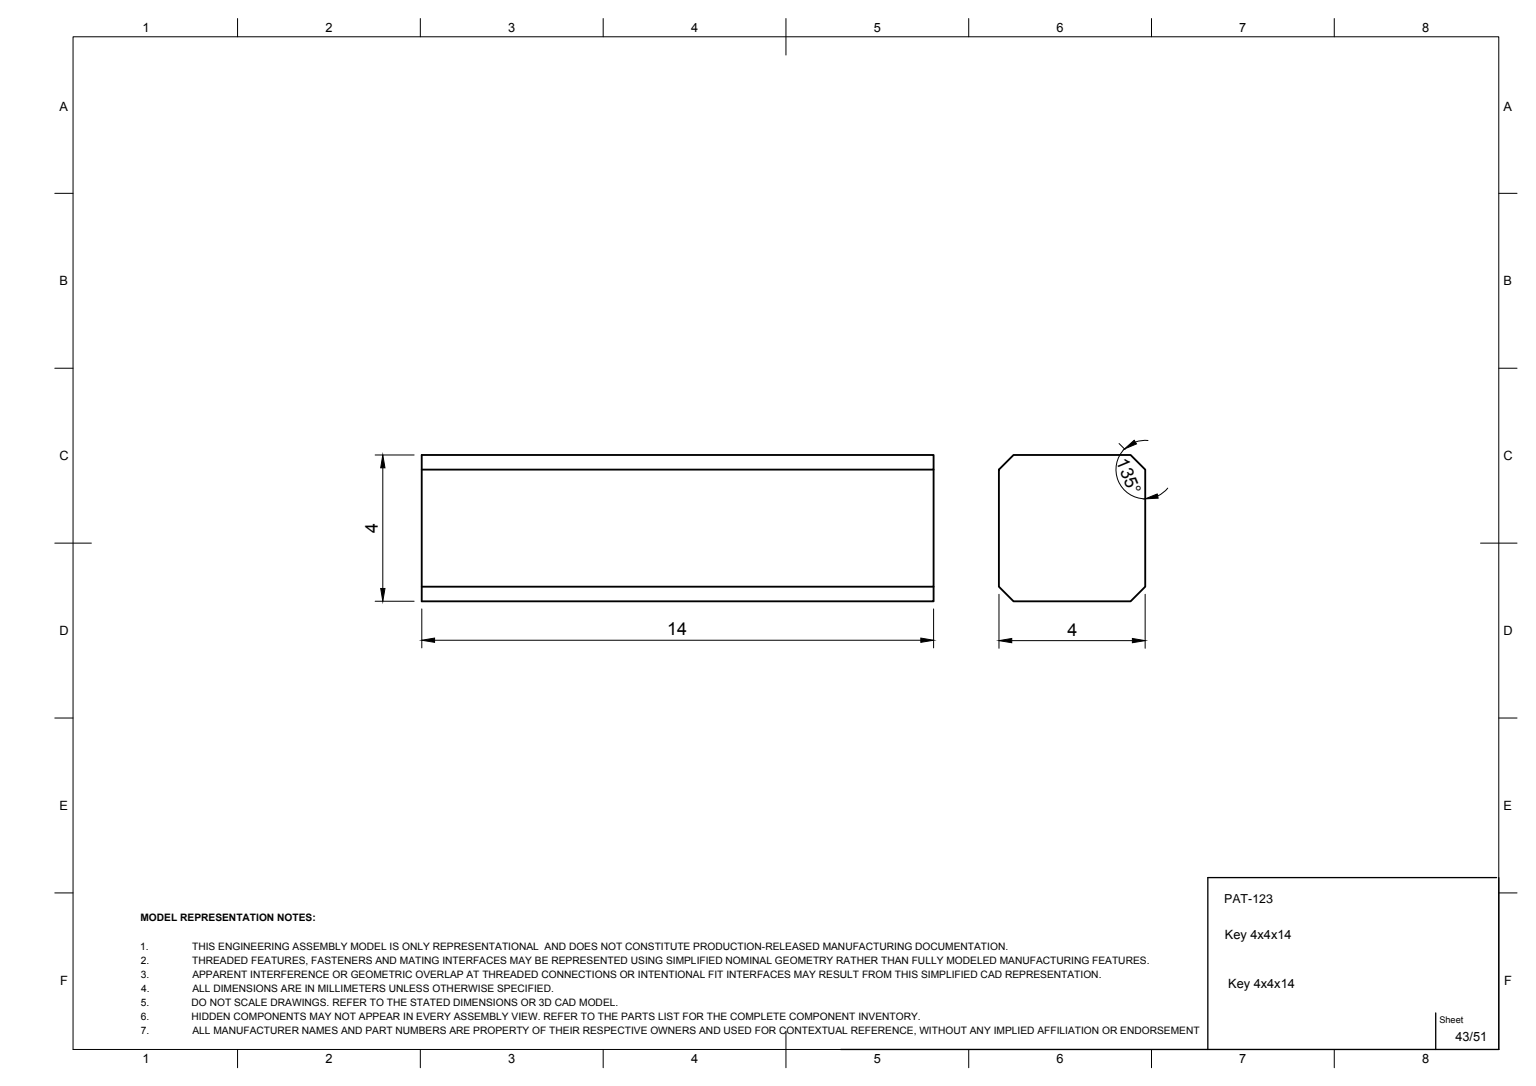
ISO-10303-21;
HEADER;
/* Generated by software containing ST-Developer
 * from STEP Tools, Inc. (www.steptools.com) 
 */

FILE_DESCRIPTION(
/* description */ ('Worm-less right-angle friction wheel drive'),
/* implementation_level */ '2;1');

FILE_NAME(
/* name */ 'Key 4x4x14.step',
/* time_stamp */ '2026-10-28T03:22:36-07:00',
/* author */ (''),
/* organization */ (''),
/* preprocessor_version */ 'ST-DEVELOPER v20.2',
/* originating_system */ 'Autodesk Translation Framework v15.17.0.0',
/* authorisation */ '');

FILE_SCHEMA (('AUTOMOTIVE_DESIGN { 1 0 10303 214 3 1 1 }'));
ENDSEC;

DATA;
#10=MECHANICAL_DESIGN_GEOMETRIC_PRESENTATION_REPRESENTATION('',(#663),#17046);
#562=SHAPE_REPRESENTATION_RELATIONSHIP('SRR','None',#17308,#609);
#609=ADVANCED_BREP_SHAPE_REPRESENTATION('',(#713),#17044);
#663=STYLED_ITEM('',(#17591),#713);
#713=MANIFOLD_SOLID_BREP('Body1',#8222);
#1189=PLANE('',#9727);
#1190=PLANE('',#9728);
#1191=PLANE('',#9729);
#1192=PLANE('',#9730);
#1193=PLANE('',#9731);
#1194=PLANE('',#9732);
#1195=PLANE('',#9733);
#1196=PLANE('',#9734);
#1197=PLANE('',#9735);
#1198=PLANE('',#9736);
#1653=FACE_OUTER_BOUND('',#2355,.T.);
#1654=FACE_OUTER_BOUND('',#2356,.T.);
#1655=FACE_OUTER_BOUND('',#2357,.T.);
#1656=FACE_OUTER_BOUND('',#2358,.T.);
#1657=FACE_OUTER_BOUND('',#2359,.T.);
#1658=FACE_OUTER_BOUND('',#2360,.T.);
#1659=FACE_OUTER_BOUND('',#2361,.T.);
#1660=FACE_OUTER_BOUND('',#2362,.T.);
#1661=FACE_OUTER_BOUND('',#2363,.T.);
#1662=FACE_OUTER_BOUND('',#2364,.T.);
#2355=EDGE_LOOP('',(#7436,#7437,#7438,#7439,#7440,#7441,#7442,#7443));
#2356=EDGE_LOOP('',(#7444,#7445,#7446,#7447));
#2357=EDGE_LOOP('',(#7448,#7449,#7450,#7451));
#2358=EDGE_LOOP('',(#7452,#7453,#7454,#7455));
#2359=EDGE_LOOP('',(#7456,#7457,#7458,#7459));
#2360=EDGE_LOOP('',(#7460,#7461,#7462,#7463,#7464,#7465,#7466,#7467));
#2361=EDGE_LOOP('',(#7468,#7469,#7470,#7471));
#2362=EDGE_LOOP('',(#7472,#7473,#7474,#7475));
#2363=EDGE_LOOP('',(#7476,#7477,#7478,#7479));
#2364=EDGE_LOOP('',(#7480,#7481,#7482,#7483));
#2873=LINE('',#16823,#3413);
#2874=LINE('',#16825,#3414);
#2875=LINE('',#16827,#3415);
#2876=LINE('',#16829,#3416);
#2877=LINE('',#16831,#3417);
#2878=LINE('',#16833,#3418);
#2879=LINE('',#16835,#3419);
#2880=LINE('',#16836,#3420);
#2881=LINE('',#16839,#3421);
#2882=LINE('',#16841,#3422);
#2883=LINE('',#16842,#3423);
#2884=LINE('',#16845,#3424);
#2885=LINE('',#16846,#3425);
#2886=LINE('',#16849,#3426);
#2887=LINE('',#16850,#3427);
#2888=LINE('',#16853,#3428);
#2889=LINE('',#16854,#3429);
#2890=LINE('',#16857,#3430);
#2891=LINE('',#16859,#3431);
#2892=LINE('',#16861,#3432);
#2893=LINE('',#16862,#3433);
#2894=LINE('',#16864,#3434);
#2895=LINE('',#16866,#3435);
#2896=LINE('',#16868,#3436);
#3413=VECTOR('',#12241,1.);
#3414=VECTOR('',#12242,1.);
#3415=VECTOR('',#12243,1.);
#3416=VECTOR('',#12244,1.);
#3417=VECTOR('',#12245,1.);
#3418=VECTOR('',#12246,1.);
#3419=VECTOR('',#12247,1.);
#3420=VECTOR('',#12248,1.);
#3421=VECTOR('',#12251,1.);
#3422=VECTOR('',#12252,1.);
#3423=VECTOR('',#12253,1.);
#3424=VECTOR('',#12256,1.);
#3425=VECTOR('',#12257,1.);
#3426=VECTOR('',#12260,1.);
#3427=VECTOR('',#12261,1.);
#3428=VECTOR('',#12264,1.);
#3429=VECTOR('',#12265,1.);
#3430=VECTOR('',#12268,1.);
#3431=VECTOR('',#12269,1.);
#3432=VECTOR('',#12270,1.);
#3433=VECTOR('',#12271,1.);
#3434=VECTOR('',#12274,1.);
#3435=VECTOR('',#12277,1.);
#3436=VECTOR('',#12280,1.);
#4505=VERTEX_POINT('',#16821);
#4506=VERTEX_POINT('',#16822);
#4507=VERTEX_POINT('',#16824);
#4508=VERTEX_POINT('',#16826);
#4509=VERTEX_POINT('',#16828);
#4510=VERTEX_POINT('',#16830);
#4511=VERTEX_POINT('',#16832);
#4512=VERTEX_POINT('',#16834);
#4513=VERTEX_POINT('',#16838);
#4514=VERTEX_POINT('',#16840);
#4515=VERTEX_POINT('',#16844);
#4516=VERTEX_POINT('',#16848);
#4517=VERTEX_POINT('',#16852);
#4518=VERTEX_POINT('',#16856);
#4519=VERTEX_POINT('',#16858);
#4520=VERTEX_POINT('',#16860);
#5487=EDGE_CURVE('',#4505,#4506,#2873,.T.);
#5488=EDGE_CURVE('',#4507,#4505,#2874,.T.);
#5489=EDGE_CURVE('',#4508,#4507,#2875,.T.);
#5490=EDGE_CURVE('',#4509,#4508,#2876,.T.);
#5491=EDGE_CURVE('',#4510,#4509,#2877,.T.);
#5492=EDGE_CURVE('',#4511,#4510,#2878,.T.);
#5493=EDGE_CURVE('',#4512,#4511,#2879,.T.);
#5494=EDGE_CURVE('',#4506,#4512,#2880,.T.);
#5495=EDGE_CURVE('',#4509,#4513,#2881,.T.);
#5496=EDGE_CURVE('',#4513,#4514,#2882,.T.);
#5497=EDGE_CURVE('',#4514,#4510,#2883,.T.);
#5498=EDGE_CURVE('',#4515,#4508,#2884,.T.);
#5499=EDGE_CURVE('',#4515,#4513,#2885,.T.);
#5500=EDGE_CURVE('',#4507,#4516,#2886,.T.);
#5501=EDGE_CURVE('',#4516,#4515,#2887,.T.);
#5502=EDGE_CURVE('',#4517,#4505,#2888,.T.);
#5503=EDGE_CURVE('',#4517,#4516,#2889,.T.);
#5504=EDGE_CURVE('',#4518,#4517,#2890,.T.);
#5505=EDGE_CURVE('',#4519,#4518,#2891,.T.);
#5506=EDGE_CURVE('',#4520,#4519,#2892,.T.);
#5507=EDGE_CURVE('',#4514,#4520,#2893,.T.);
#5508=EDGE_CURVE('',#4506,#4518,#2894,.T.);
#5509=EDGE_CURVE('',#4519,#4512,#2895,.T.);
#5510=EDGE_CURVE('',#4511,#4520,#2896,.T.);
#7436=ORIENTED_EDGE('',*,*,#5487,.F.);
#7437=ORIENTED_EDGE('',*,*,#5488,.F.);
#7438=ORIENTED_EDGE('',*,*,#5489,.F.);
#7439=ORIENTED_EDGE('',*,*,#5490,.F.);
#7440=ORIENTED_EDGE('',*,*,#5491,.F.);
#7441=ORIENTED_EDGE('',*,*,#5492,.F.);
#7442=ORIENTED_EDGE('',*,*,#5493,.F.);
#7443=ORIENTED_EDGE('',*,*,#5494,.F.);
#7444=ORIENTED_EDGE('',*,*,#5491,.T.);
#7445=ORIENTED_EDGE('',*,*,#5495,.T.);
#7446=ORIENTED_EDGE('',*,*,#5496,.T.);
#7447=ORIENTED_EDGE('',*,*,#5497,.T.);
#7448=ORIENTED_EDGE('',*,*,#5490,.T.);
#7449=ORIENTED_EDGE('',*,*,#5498,.F.);
#7450=ORIENTED_EDGE('',*,*,#5499,.T.);
#7451=ORIENTED_EDGE('',*,*,#5495,.F.);
#7452=ORIENTED_EDGE('',*,*,#5489,.T.);
#7453=ORIENTED_EDGE('',*,*,#5500,.T.);
#7454=ORIENTED_EDGE('',*,*,#5501,.T.);
#7455=ORIENTED_EDGE('',*,*,#5498,.T.);
#7456=ORIENTED_EDGE('',*,*,#5488,.T.);
#7457=ORIENTED_EDGE('',*,*,#5502,.F.);
#7458=ORIENTED_EDGE('',*,*,#5503,.T.);
#7459=ORIENTED_EDGE('',*,*,#5500,.F.);
#7460=ORIENTED_EDGE('',*,*,#5496,.F.);
#7461=ORIENTED_EDGE('',*,*,#5499,.F.);
#7462=ORIENTED_EDGE('',*,*,#5501,.F.);
#7463=ORIENTED_EDGE('',*,*,#5503,.F.);
#7464=ORIENTED_EDGE('',*,*,#5504,.F.);
#7465=ORIENTED_EDGE('',*,*,#5505,.F.);
#7466=ORIENTED_EDGE('',*,*,#5506,.F.);
#7467=ORIENTED_EDGE('',*,*,#5507,.F.);
#7468=ORIENTED_EDGE('',*,*,#5487,.T.);
#7469=ORIENTED_EDGE('',*,*,#5508,.T.);
#7470=ORIENTED_EDGE('',*,*,#5504,.T.);
#7471=ORIENTED_EDGE('',*,*,#5502,.T.);
#7472=ORIENTED_EDGE('',*,*,#5494,.T.);
#7473=ORIENTED_EDGE('',*,*,#5509,.F.);
#7474=ORIENTED_EDGE('',*,*,#5505,.T.);
#7475=ORIENTED_EDGE('',*,*,#5508,.F.);
#7476=ORIENTED_EDGE('',*,*,#5493,.T.);
#7477=ORIENTED_EDGE('',*,*,#5510,.T.);
#7478=ORIENTED_EDGE('',*,*,#5506,.T.);
#7479=ORIENTED_EDGE('',*,*,#5509,.T.);
#7480=ORIENTED_EDGE('',*,*,#5492,.T.);
#7481=ORIENTED_EDGE('',*,*,#5497,.F.);
#7482=ORIENTED_EDGE('',*,*,#5507,.T.);
#7483=ORIENTED_EDGE('',*,*,#5510,.F.);
#8145=ADVANCED_FACE('',(#1653),#1189,.T.);
#8146=ADVANCED_FACE('',(#1654),#1190,.T.);
#8147=ADVANCED_FACE('',(#1655),#1191,.T.);
#8148=ADVANCED_FACE('',(#1656),#1192,.T.);
#8149=ADVANCED_FACE('',(#1657),#1193,.T.);
#8150=ADVANCED_FACE('',(#1658),#1194,.F.);
#8151=ADVANCED_FACE('',(#1659),#1195,.T.);
#8152=ADVANCED_FACE('',(#1660),#1196,.T.);
#8153=ADVANCED_FACE('',(#1661),#1197,.T.);
#8154=ADVANCED_FACE('',(#1662),#1198,.F.);
#8222=CLOSED_SHELL('',(#8145,#8146,#8147,#8148,#8149,#8150,#8151,#8152,
#8153,#8154));
#9726=AXIS2_PLACEMENT_3D('',#16819,#12237,#12238);
#9727=AXIS2_PLACEMENT_3D('',#16820,#12239,#12240);
#9728=AXIS2_PLACEMENT_3D('',#16837,#12249,#12250);
#9729=AXIS2_PLACEMENT_3D('',#16843,#12254,#12255);
#9730=AXIS2_PLACEMENT_3D('',#16847,#12258,#12259);
#9731=AXIS2_PLACEMENT_3D('',#16851,#12262,#12263);
#9732=AXIS2_PLACEMENT_3D('',#16855,#12266,#12267);
#9733=AXIS2_PLACEMENT_3D('',#16863,#12272,#12273);
#9734=AXIS2_PLACEMENT_3D('',#16865,#12275,#12276);
#9735=AXIS2_PLACEMENT_3D('',#16867,#12278,#12279);
#9736=AXIS2_PLACEMENT_3D('',#16869,#12281,#12282);
#12237=DIRECTION('axis',(0.,0.,1.));
#12238=DIRECTION('refdir',(1.,0.,0.));
#12239=DIRECTION('center_axis',(1.,0.,0.));
#12240=DIRECTION('ref_axis',(0.,0.,-1.));
#12241=DIRECTION('',(0.,0.707106781186547,-0.707106781186548));
#12242=DIRECTION('',(0.,1.,0.));
#12243=DIRECTION('',(0.,0.707106781186547,0.707106781186548));
#12244=DIRECTION('',(0.,0.,1.));
#12245=DIRECTION('',(0.,-0.707106781186548,0.707106781186548));
#12246=DIRECTION('',(0.,-1.,0.));
#12247=DIRECTION('',(0.,-0.707106781186548,-0.707106781186548));
#12248=DIRECTION('',(0.,0.,-1.));
#12249=DIRECTION('center_axis',(0.,-0.707106781186548,-0.707106781186548));
#12250=DIRECTION('ref_axis',(-1.,0.,0.));
#12251=DIRECTION('',(-1.,0.,0.));
#12252=DIRECTION('',(0.,0.707106781186548,-0.707106781186548));
#12253=DIRECTION('',(1.,0.,0.));
#12254=DIRECTION('center_axis',(0.,-1.,0.));
#12255=DIRECTION('ref_axis',(1.,0.,0.));
#12256=DIRECTION('',(1.,0.,0.));
#12257=DIRECTION('',(0.,0.,-1.));
#12258=DIRECTION('center_axis',(0.,-0.707106781186548,0.707106781186547));
#12259=DIRECTION('ref_axis',(1.,0.,0.));
#12260=DIRECTION('',(-1.,0.,0.));
#12261=DIRECTION('',(0.,-0.707106781186547,-0.707106781186548));
#12262=DIRECTION('center_axis',(0.,0.,1.));
#12263=DIRECTION('ref_axis',(1.,0.,0.));
#12264=DIRECTION('',(1.,0.,0.));
#12265=DIRECTION('',(0.,-1.,0.));
#12266=DIRECTION('center_axis',(1.,0.,0.));
#12267=DIRECTION('ref_axis',(0.,0.,-1.));
#12268=DIRECTION('',(0.,-0.707106781186547,0.707106781186548));
#12269=DIRECTION('',(0.,0.,1.));
#12270=DIRECTION('',(0.,0.707106781186548,0.707106781186548));
#12271=DIRECTION('',(0.,1.,0.));
#12272=DIRECTION('center_axis',(0.,0.707106781186548,0.707106781186547));
#12273=DIRECTION('ref_axis',(1.,0.,0.));
#12274=DIRECTION('',(-1.,0.,0.));
#12275=DIRECTION('center_axis',(0.,1.,0.));
#12276=DIRECTION('ref_axis',(-1.,0.,0.));
#12277=DIRECTION('',(1.,0.,0.));
#12278=DIRECTION('center_axis',(0.,0.707106781186548,-0.707106781186548));
#12279=DIRECTION('ref_axis',(-1.,0.,0.));
#12280=DIRECTION('',(-1.,0.,0.));
#12281=DIRECTION('center_axis',(0.,0.,1.));
#12282=DIRECTION('ref_axis',(1.,0.,0.));
#16819=CARTESIAN_POINT('',(0.,0.,0.));
#16820=CARTESIAN_POINT('Origin',(0.7,0.,0.25));
#16821=CARTESIAN_POINT('',(0.7,0.16,0.4));
#16822=CARTESIAN_POINT('',(0.7,0.2,0.36));
#16823=CARTESIAN_POINT('',(0.7,0.1675,0.3925));
#16824=CARTESIAN_POINT('',(0.7,-0.16,0.4));
#16825=CARTESIAN_POINT('',(0.7,0.,0.4));
#16826=CARTESIAN_POINT('',(0.7,-0.2,0.36));
#16827=CARTESIAN_POINT('',(0.7,-0.1675,0.3925));
#16828=CARTESIAN_POINT('',(0.7,-0.2,0.04));
#16829=CARTESIAN_POINT('',(0.7,-0.2,0.125));
#16830=CARTESIAN_POINT('',(0.7,-0.16,0.));
#16831=CARTESIAN_POINT('',(0.7,-0.1925,0.0325));
#16832=CARTESIAN_POINT('',(0.7,0.16,0.));
#16833=CARTESIAN_POINT('',(0.7,0.,0.));
#16834=CARTESIAN_POINT('',(0.7,0.2,0.04));
#16835=CARTESIAN_POINT('',(0.7,0.1925,0.0325));
#16836=CARTESIAN_POINT('',(0.7,0.2,0.125));
#16837=CARTESIAN_POINT('Origin',(-0.4,-0.18,0.02));
#16838=CARTESIAN_POINT('',(-0.7,-0.2,0.04));
#16839=CARTESIAN_POINT('',(-0.4,-0.2,0.04));
#16840=CARTESIAN_POINT('',(-0.7,-0.16,0.));
#16841=CARTESIAN_POINT('',(-0.7,-0.1925,0.0325));
#16842=CARTESIAN_POINT('',(-0.4,-0.16,0.));
#16843=CARTESIAN_POINT('Origin',(-0.8,-0.2,0.));
#16844=CARTESIAN_POINT('',(-0.7,-0.2,0.36));
#16845=CARTESIAN_POINT('',(-0.4,-0.2,0.36));
#16846=CARTESIAN_POINT('',(-0.7,-0.2,0.125));
#16847=CARTESIAN_POINT('Origin',(-0.4,-0.18,0.38));
#16848=CARTESIAN_POINT('',(-0.7,-0.16,0.4));
#16849=CARTESIAN_POINT('',(-0.4,-0.16,0.4));
#16850=CARTESIAN_POINT('',(-0.7,-0.1675,0.3925));
#16851=CARTESIAN_POINT('Origin',(0.,0.,0.4));
#16852=CARTESIAN_POINT('',(-0.7,0.16,0.4));
#16853=CARTESIAN_POINT('',(0.4,0.16,0.4));
#16854=CARTESIAN_POINT('',(-0.7,0.,0.4));
#16855=CARTESIAN_POINT('Origin',(-0.7,0.,0.25));
#16856=CARTESIAN_POINT('',(-0.7,0.2,0.36));
#16857=CARTESIAN_POINT('',(-0.7,0.1675,0.3925));
#16858=CARTESIAN_POINT('',(-0.7,0.2,0.04));
#16859=CARTESIAN_POINT('',(-0.7,0.2,0.125));
#16860=CARTESIAN_POINT('',(-0.7,0.16,0.));
#16861=CARTESIAN_POINT('',(-0.7,0.1925,0.0325));
#16862=CARTESIAN_POINT('',(-0.7,0.,0.));
#16863=CARTESIAN_POINT('Origin',(0.4,0.18,0.38));
#16864=CARTESIAN_POINT('',(0.4,0.2,0.36));
#16865=CARTESIAN_POINT('Origin',(0.8,0.2,0.));
#16866=CARTESIAN_POINT('',(0.4,0.2,0.04));
#16867=CARTESIAN_POINT('Origin',(0.4,0.18,0.02));
#16868=CARTESIAN_POINT('',(0.4,0.16,0.));
#16869=CARTESIAN_POINT('Origin',(0.,0.,0.));
#16991=UNCERTAINTY_MEASURE_WITH_UNIT(LENGTH_MEASURE(0.001),#17047,
'DISTANCE_ACCURACY_VALUE',
'Maximum model space distance between geometric entities at asserted c
onnectivities');
#16993=UNCERTAINTY_MEASURE_WITH_UNIT(LENGTH_MEASURE(0.001),#17047,
'DISTANCE_ACCURACY_VALUE',
'Maximum model space distance between geometric entities at asserted c
onnectivities');
#17044=(
GEOMETRIC_REPRESENTATION_CONTEXT(3)
GLOBAL_UNCERTAINTY_ASSIGNED_CONTEXT((#16991))
GLOBAL_UNIT_ASSIGNED_CONTEXT((#17047,#17049,#17050))
REPRESENTATION_CONTEXT('','3D')
);
#17046=(
GEOMETRIC_REPRESENTATION_CONTEXT(3)
GLOBAL_UNCERTAINTY_ASSIGNED_CONTEXT((#16993))
GLOBAL_UNIT_ASSIGNED_CONTEXT((#17047,#17049,#17050))
REPRESENTATION_CONTEXT('','3D')
);
#17047=(
LENGTH_UNIT()
NAMED_UNIT(*)
SI_UNIT(.CENTI.,.METRE.)
);
#17049=(
NAMED_UNIT(*)
PLANE_ANGLE_UNIT()
SI_UNIT($,.RADIAN.)
);
#17050=(
NAMED_UNIT(*)
SI_UNIT($,.STERADIAN.)
SOLID_ANGLE_UNIT()
);
#17101=SHAPE_DEFINITION_REPRESENTATION(#17235,#17308);
#17235=PRODUCT_DEFINITION_SHAPE('',$,#17361);
#17308=SHAPE_REPRESENTATION('',(#9726),#17044);
#17310=PRODUCT_DEFINITION_CONTEXT('part definition',#17468,'design');
#17361=PRODUCT_DEFINITION('Key 4x4x14','Key 4x4x14',#17413,#17310);
#17413=PRODUCT_DEFINITION_FORMATION('',$,#17520);
#17468=APPLICATION_CONTEXT(
'Core Data for Automotive Mechanical Design Process');
#17469=PRODUCT_CONTEXT('part definition',#17468,'mechanical');
#17520=PRODUCT('Key 4x4x14','Key 4x4x14','Key 4x4x14',(#17469));
#17585=COLOUR_RGB('Grey',0.48,0.52,0.57);
#17586=FILL_AREA_STYLE_COLOUR('',#17585);
#17587=FILL_AREA_STYLE('',(#17586));
#17588=SURFACE_STYLE_FILL_AREA(#17587);
#17589=SURFACE_SIDE_STYLE('',(#17588));
#17590=SURFACE_STYLE_USAGE(.BOTH.,#17589);
#17591=PRESENTATION_STYLE_ASSIGNMENT((#17590));
ENDSEC;
END-ISO-10303-21;
